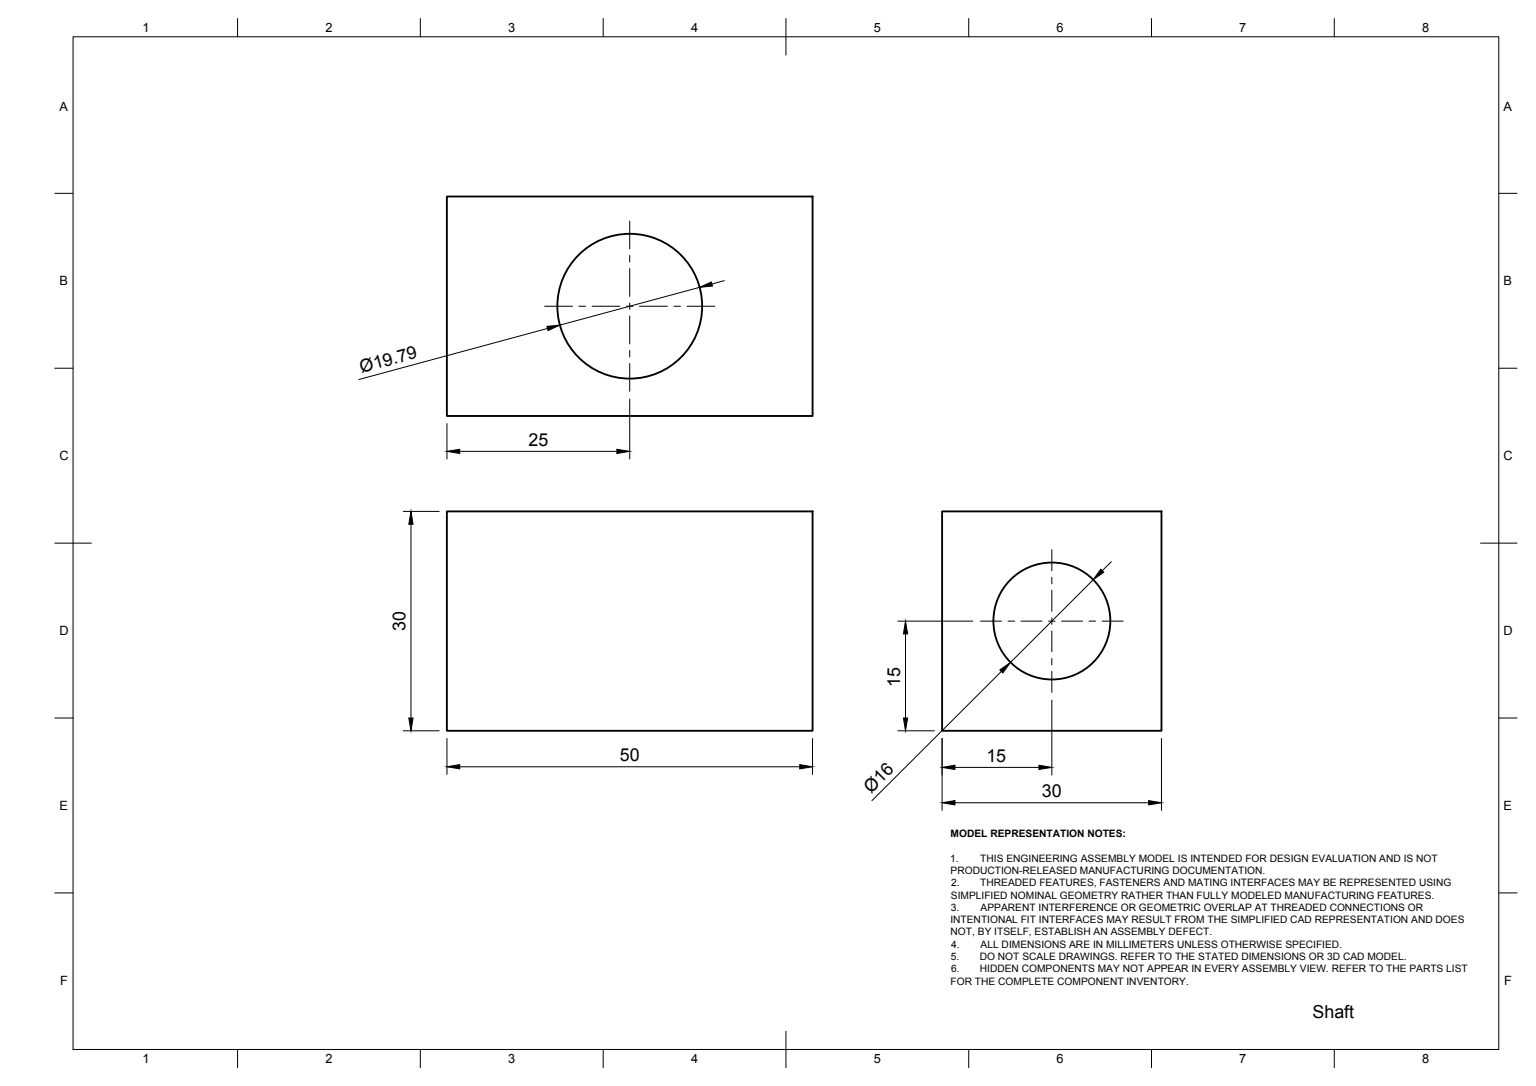
ISO-10303-21;
HEADER;
/* Generated by software containing ST-Developer
 * from STEP Tools, Inc. (www.steptools.com) 
 */

FILE_DESCRIPTION(
/* description */ (''),
/* implementation_level */ '2;1');

FILE_NAME(
/* name */ 'Shaft.step',
/* time_stamp */ '2026-10-05T19:45:59-07:00',
/* author */ (''),
/* organization */ (''),
/* preprocessor_version */ 'ST-DEVELOPER v20.2',
/* originating_system */ 'Autodesk Translation Framework v15.15.0.0',
/* authorisation */ '');

FILE_SCHEMA (('AUTOMOTIVE_DESIGN { 1 0 10303 214 3 1 1 }'));
ENDSEC;

DATA;
#10=MECHANICAL_DESIGN_GEOMETRIC_PRESENTATION_REPRESENTATION('',(#96),#2462);
#52=B_SPLINE_CURVE_WITH_KNOTS('',3,(#2172,#2173,#2174,#2175,#2176,#2177,
#2178,#2179,#2180,#2181,#2182,#2183,#2184,#2185,#2186,#2187,#2188,#2189,
#2190,#2191,#2192,#2193),.UNSPECIFIED.,.F.,.F.,(4,2,2,2,2,2,2,2,2,2,4),
(1.29528463060384,1.61362869954164,1.93197276847945,2.26127101484344,2.42592013802544,
2.59056926120743,2.75521838438943,2.91986750757142,3.24916575393542,3.56750982287322,
3.88585389181102),.UNSPECIFIED.);
#53=B_SPLINE_CURVE_WITH_KNOTS('',3,(#2198,#2199,#2200,#2201,#2202,#2203,
#2204,#2205,#2206,#2207,#2208,#2209),.UNSPECIFIED.,.F.,.F.,(4,2,2,2,2,4),
(0.,0.164649123182026,0.329298246364052,0.658596492728105,0.976940561665974,
1.29528463060384),.UNSPECIFIED.);
#54=B_SPLINE_CURVE_WITH_KNOTS('',3,(#2210,#2211,#2212,#2213,#2214,#2215,
#2216,#2217,#2218,#2219,#2220,#2221),.UNSPECIFIED.,.F.,.F.,(4,2,2,2,2,4),
(3.88585389181102,4.20419796074889,4.52254202968676,4.85184027605081,5.01648939923284,
5.18113852241487),.UNSPECIFIED.);
#55=B_SPLINE_CURVE_WITH_KNOTS('',3,(#2223,#2224,#2225,#2226,#2227,#2228,
#2229,#2230,#2231,#2232,#2233,#2234,#2235,#2236,#2237,#2238,#2239,#2240,
#2241,#2242,#2243,#2244,#2245,#2246,#2247,#2248,#2249,#2250,#2251,#2252,
#2253,#2254,#2255,#2256,#2257,#2258,#2259,#2260,#2261,#2262,#2263,#2264),
 .UNSPECIFIED.,.T.,.F.,(4,2,2,2,2,2,2,2,2,2,2,2,2,2,2,2,2,2,2,2,4),(0.,
0.164649123182026,0.329298246364052,0.658596492728105,0.976940561665974,
1.29528463060384,1.61362869954165,1.93197276847945,2.26127101484344,2.42592013802544,
2.59056926120743,2.75521838438943,2.91986750757143,3.24916575393542,3.56750982287322,
3.88585389181102,4.20419796074889,4.52254202968676,4.85184027605081,5.01648939923284,
5.18113852241487),.UNSPECIFIED.);
#65=FACE_BOUND('',#295,.T.);
#66=FACE_BOUND('',#298,.T.);
#67=FACE_BOUND('',#302,.T.);
#68=FACE_BOUND('',#305,.T.);
#69=FACE_BOUND('',#307,.T.);
#78=SHAPE_REPRESENTATION_RELATIONSHIP('SRR','None',#2504,#87);
#87=ADVANCED_BREP_SHAPE_REPRESENTATION('',(#105),#2459);
#96=STYLED_ITEM('',(#2552),#105);
#105=MANIFOLD_SOLID_BREP('Body1',#1333);
#136=PLANE('',#1515);
#137=PLANE('',#1518);
#138=PLANE('',#1519);
#139=PLANE('',#1520);
#140=PLANE('',#1521);
#141=PLANE('',#1522);
#206=FACE_OUTER_BOUND('',#294,.T.);
#207=FACE_OUTER_BOUND('',#296,.T.);
#208=FACE_OUTER_BOUND('',#297,.T.);
#209=FACE_OUTER_BOUND('',#299,.T.);
#210=FACE_OUTER_BOUND('',#300,.T.);
#211=FACE_OUTER_BOUND('',#301,.T.);
#212=FACE_OUTER_BOUND('',#303,.T.);
#213=FACE_OUTER_BOUND('',#304,.T.);
#214=FACE_OUTER_BOUND('',#306,.T.);
#294=EDGE_LOOP('',(#1054,#1055,#1056,#1057,#1058,#1059,#1060,#1061,#1062));
#295=EDGE_LOOP('',(#1063));
#296=EDGE_LOOP('',(#1064,#1065,#1066,#1067,#1068,#1069));
#297=EDGE_LOOP('',(#1070,#1071,#1072,#1073));
#298=EDGE_LOOP('',(#1074));
#299=EDGE_LOOP('',(#1075,#1076,#1077,#1078));
#300=EDGE_LOOP('',(#1079,#1080,#1081,#1082));
#301=EDGE_LOOP('',(#1083,#1084,#1085,#1086));
#302=EDGE_LOOP('',(#1087));
#303=EDGE_LOOP('',(#1088,#1089,#1090,#1091));
#304=EDGE_LOOP('',(#1092,#1093,#1094,#1095));
#305=EDGE_LOOP('',(#1096));
#306=EDGE_LOOP('',(#1097,#1098,#1099,#1100));
#307=EDGE_LOOP('',(#1101));
#395=LINE('',#2170,#514);
#396=LINE('',#2195,#515);
#397=LINE('',#2268,#516);
#398=LINE('',#2272,#517);
#399=LINE('',#2274,#518);
#400=LINE('',#2276,#519);
#401=LINE('',#2277,#520);
#402=LINE('',#2280,#521);
#403=LINE('',#2284,#522);
#404=LINE('',#2286,#523);
#405=LINE('',#2287,#524);
#406=LINE('',#2290,#525);
#407=LINE('',#2291,#526);
#408=LINE('',#2294,#527);
#409=LINE('',#2295,#528);
#410=LINE('',#2297,#529);
#514=VECTOR('',#1786,9.89525);
#515=VECTOR('',#1787,9.89525);
#516=VECTOR('',#1794,8.);
#517=VECTOR('',#1797,10.);
#518=VECTOR('',#1798,10.);
#519=VECTOR('',#1799,10.);
#520=VECTOR('',#1800,10.);
#521=VECTOR('',#1803,8.);
#522=VECTOR('',#1808,10.);
#523=VECTOR('',#1809,10.);
#524=VECTOR('',#1810,10.);
#525=VECTOR('',#1813,10.);
#526=VECTOR('',#1814,10.);
#527=VECTOR('',#1817,10.);
#528=VECTOR('',#1818,10.);
#529=VECTOR('',#1821,10.);
#603=CIRCLE('',#1511,9.89525);
#604=CIRCLE('',#1512,9.89525);
#605=CIRCLE('',#1514,8.);
#606=CIRCLE('',#1517,8.);
#674=VERTEX_POINT('',#2167);
#675=VERTEX_POINT('',#2169);
#676=VERTEX_POINT('',#2171);
#677=VERTEX_POINT('',#2194);
#678=VERTEX_POINT('',#2197);
#679=VERTEX_POINT('',#2222);
#680=VERTEX_POINT('',#2266);
#681=VERTEX_POINT('',#2270);
#682=VERTEX_POINT('',#2271);
#683=VERTEX_POINT('',#2273);
#684=VERTEX_POINT('',#2275);
#685=VERTEX_POINT('',#2279);
#686=VERTEX_POINT('',#2283);
#687=VERTEX_POINT('',#2285);
#688=VERTEX_POINT('',#2289);
#689=VERTEX_POINT('',#2293);
#808=EDGE_CURVE('',#674,#674,#603,.T.);
#809=EDGE_CURVE('',#674,#675,#395,.T.);
#810=EDGE_CURVE('',#676,#675,#52,.T.);
#811=EDGE_CURVE('',#676,#677,#396,.T.);
#812=EDGE_CURVE('',#677,#677,#604,.T.);
#813=EDGE_CURVE('',#678,#676,#53,.T.);
#814=EDGE_CURVE('',#675,#678,#54,.T.);
#815=EDGE_CURVE('',#679,#679,#55,.T.);
#816=EDGE_CURVE('',#680,#680,#605,.T.);
#817=EDGE_CURVE('',#680,#678,#397,.T.);
#818=EDGE_CURVE('',#681,#682,#398,.T.);
#819=EDGE_CURVE('',#682,#683,#399,.T.);
#820=EDGE_CURVE('',#683,#684,#400,.T.);
#821=EDGE_CURVE('',#684,#681,#401,.T.);
#822=EDGE_CURVE('',#679,#685,#402,.T.);
#823=EDGE_CURVE('',#685,#685,#606,.T.);
#824=EDGE_CURVE('',#686,#682,#403,.T.);
#825=EDGE_CURVE('',#687,#686,#404,.T.);
#826=EDGE_CURVE('',#683,#687,#405,.T.);
#827=EDGE_CURVE('',#688,#687,#406,.T.);
#828=EDGE_CURVE('',#684,#688,#407,.T.);
#829=EDGE_CURVE('',#689,#688,#408,.T.);
#830=EDGE_CURVE('',#681,#689,#409,.T.);
#831=EDGE_CURVE('',#686,#689,#410,.T.);
#1054=ORIENTED_EDGE('',*,*,#808,.F.);
#1055=ORIENTED_EDGE('',*,*,#809,.T.);
#1056=ORIENTED_EDGE('',*,*,#810,.F.);
#1057=ORIENTED_EDGE('',*,*,#811,.T.);
#1058=ORIENTED_EDGE('',*,*,#812,.F.);
#1059=ORIENTED_EDGE('',*,*,#811,.F.);
#1060=ORIENTED_EDGE('',*,*,#813,.F.);
#1061=ORIENTED_EDGE('',*,*,#814,.F.);
#1062=ORIENTED_EDGE('',*,*,#809,.F.);
#1063=ORIENTED_EDGE('',*,*,#815,.F.);
#1064=ORIENTED_EDGE('',*,*,#816,.F.);
#1065=ORIENTED_EDGE('',*,*,#817,.T.);
#1066=ORIENTED_EDGE('',*,*,#813,.T.);
#1067=ORIENTED_EDGE('',*,*,#810,.T.);
#1068=ORIENTED_EDGE('',*,*,#814,.T.);
#1069=ORIENTED_EDGE('',*,*,#817,.F.);
#1070=ORIENTED_EDGE('',*,*,#818,.T.);
#1071=ORIENTED_EDGE('',*,*,#819,.T.);
#1072=ORIENTED_EDGE('',*,*,#820,.T.);
#1073=ORIENTED_EDGE('',*,*,#821,.T.);
#1074=ORIENTED_EDGE('',*,*,#816,.T.);
#1075=ORIENTED_EDGE('',*,*,#815,.T.);
#1076=ORIENTED_EDGE('',*,*,#822,.T.);
#1077=ORIENTED_EDGE('',*,*,#823,.F.);
#1078=ORIENTED_EDGE('',*,*,#822,.F.);
#1079=ORIENTED_EDGE('',*,*,#824,.F.);
#1080=ORIENTED_EDGE('',*,*,#825,.F.);
#1081=ORIENTED_EDGE('',*,*,#826,.F.);
#1082=ORIENTED_EDGE('',*,*,#819,.F.);
#1083=ORIENTED_EDGE('',*,*,#826,.T.);
#1084=ORIENTED_EDGE('',*,*,#827,.F.);
#1085=ORIENTED_EDGE('',*,*,#828,.F.);
#1086=ORIENTED_EDGE('',*,*,#820,.F.);
#1087=ORIENTED_EDGE('',*,*,#812,.T.);
#1088=ORIENTED_EDGE('',*,*,#828,.T.);
#1089=ORIENTED_EDGE('',*,*,#829,.F.);
#1090=ORIENTED_EDGE('',*,*,#830,.F.);
#1091=ORIENTED_EDGE('',*,*,#821,.F.);
#1092=ORIENTED_EDGE('',*,*,#830,.T.);
#1093=ORIENTED_EDGE('',*,*,#831,.F.);
#1094=ORIENTED_EDGE('',*,*,#824,.T.);
#1095=ORIENTED_EDGE('',*,*,#818,.F.);
#1096=ORIENTED_EDGE('',*,*,#808,.T.);
#1097=ORIENTED_EDGE('',*,*,#831,.T.);
#1098=ORIENTED_EDGE('',*,*,#829,.T.);
#1099=ORIENTED_EDGE('',*,*,#827,.T.);
#1100=ORIENTED_EDGE('',*,*,#825,.T.);
#1101=ORIENTED_EDGE('',*,*,#823,.T.);
#1238=CYLINDRICAL_SURFACE('',#1510,9.89525);
#1239=CYLINDRICAL_SURFACE('',#1513,8.);
#1240=CYLINDRICAL_SURFACE('',#1516,8.);
#1288=ADVANCED_FACE('',(#206,#65),#1238,.F.);
#1289=ADVANCED_FACE('',(#207),#1239,.F.);
#1290=ADVANCED_FACE('',(#208,#66),#136,.F.);
#1291=ADVANCED_FACE('',(#209),#1240,.F.);
#1292=ADVANCED_FACE('',(#210),#137,.T.);
#1293=ADVANCED_FACE('',(#211,#67),#138,.T.);
#1294=ADVANCED_FACE('',(#212),#139,.T.);
#1295=ADVANCED_FACE('',(#213,#68),#140,.T.);
#1296=ADVANCED_FACE('',(#214,#69),#141,.T.);
#1333=CLOSED_SHELL('',(#1288,#1289,#1290,#1291,#1292,#1293,#1294,#1295,
#1296));
#1509=AXIS2_PLACEMENT_3D('',#2165,#1780,#1781);
#1510=AXIS2_PLACEMENT_3D('',#2166,#1782,#1783);
#1511=AXIS2_PLACEMENT_3D('',#2168,#1784,#1785);
#1512=AXIS2_PLACEMENT_3D('',#2196,#1788,#1789);
#1513=AXIS2_PLACEMENT_3D('',#2265,#1790,#1791);
#1514=AXIS2_PLACEMENT_3D('',#2267,#1792,#1793);
#1515=AXIS2_PLACEMENT_3D('',#2269,#1795,#1796);
#1516=AXIS2_PLACEMENT_3D('',#2278,#1801,#1802);
#1517=AXIS2_PLACEMENT_3D('',#2281,#1804,#1805);
#1518=AXIS2_PLACEMENT_3D('',#2282,#1806,#1807);
#1519=AXIS2_PLACEMENT_3D('',#2288,#1811,#1812);
#1520=AXIS2_PLACEMENT_3D('',#2292,#1815,#1816);
#1521=AXIS2_PLACEMENT_3D('',#2296,#1819,#1820);
#1522=AXIS2_PLACEMENT_3D('',#2298,#1822,#1823);
#1780=DIRECTION('axis',(0.,0.,1.));
#1781=DIRECTION('refdir',(1.,0.,0.));
#1782=DIRECTION('center_axis',(0.,0.,-1.));
#1783=DIRECTION('ref_axis',(-1.,0.,0.));
#1784=DIRECTION('center_axis',(0.,0.,-1.));
#1785=DIRECTION('ref_axis',(-1.,0.,0.));
#1786=DIRECTION('',(0.,0.,-1.));
#1787=DIRECTION('',(0.,0.,-1.));
#1788=DIRECTION('center_axis',(0.,7.40148683083438E-17,1.));
#1789=DIRECTION('ref_axis',(-1.,0.,0.));
#1790=DIRECTION('center_axis',(-1.,0.,0.));
#1791=DIRECTION('ref_axis',(0.,-1.,0.));
#1792=DIRECTION('center_axis',(-1.,0.,0.));
#1793=DIRECTION('ref_axis',(0.,-1.,0.));
#1794=DIRECTION('',(-1.,0.,0.));
#1795=DIRECTION('center_axis',(-1.,0.,0.));
#1796=DIRECTION('ref_axis',(0.,-1.,0.));
#1797=DIRECTION('',(0.,-1.,0.));
#1798=DIRECTION('',(0.,0.,-1.));
#1799=DIRECTION('',(0.,1.,-7.40148683083438E-17));
#1800=DIRECTION('',(0.,0.,1.));
#1801=DIRECTION('center_axis',(-1.,0.,0.));
#1802=DIRECTION('ref_axis',(0.,-1.,0.));
#1803=DIRECTION('',(-1.,0.,0.));
#1804=DIRECTION('center_axis',(1.,0.,0.));
#1805=DIRECTION('ref_axis',(0.,-1.,0.));
#1806=DIRECTION('center_axis',(0.,-1.,0.));
#1807=DIRECTION('ref_axis',(0.,0.,1.));
#1808=DIRECTION('',(1.,0.,0.));
#1809=DIRECTION('',(0.,0.,1.));
#1810=DIRECTION('',(-1.,0.,0.));
#1811=DIRECTION('center_axis',(0.,-7.40148683083438E-17,-1.));
#1812=DIRECTION('ref_axis',(0.,-1.,7.40148683083438E-17));
#1813=DIRECTION('',(0.,-1.,7.40148683083438E-17));
#1814=DIRECTION('',(-1.,0.,0.));
#1815=DIRECTION('center_axis',(0.,1.,0.));
#1816=DIRECTION('ref_axis',(0.,0.,-1.));
#1817=DIRECTION('',(0.,0.,-1.));
#1818=DIRECTION('',(-1.,0.,0.));
#1819=DIRECTION('center_axis',(0.,0.,1.));
#1820=DIRECTION('ref_axis',(0.,1.,0.));
#1821=DIRECTION('',(0.,1.,0.));
#1822=DIRECTION('center_axis',(-1.,0.,0.));
#1823=DIRECTION('ref_axis',(0.,-1.,0.));
#2165=CARTESIAN_POINT('',(0.,0.,0.));
#2166=CARTESIAN_POINT('Origin',(152.4,-2.52242671194836E-12,14.9999999999958));
#2167=CARTESIAN_POINT('',(162.29525,-2.52121489332443E-12,14.9999999999958));
#2168=CARTESIAN_POINT('Origin',(152.4,-2.52242671194836E-12,14.9999999999958));
#2169=CARTESIAN_POINT('',(162.29525,-1.26161109846903E-12,8.));
#2170=CARTESIAN_POINT('',(162.29525,-2.52363853057229E-12,14.9999999999958));
#2171=CARTESIAN_POINT('',(162.29525,-1.26119476483479E-12,-8.));
#2172=CARTESIAN_POINT('Ctrl Pts',(162.29525,1.66533453693773E-15,-8.));
#2173=CARTESIAN_POINT('Ctrl Pts',(162.29525,-1.06114689645934,-8.));
#2174=CARTESIAN_POINT('Ctrl Pts',(162.112073508216,-2.15862639679729,-7.77661292309447));
#2175=CARTESIAN_POINT('Ctrl Pts',(161.456447542343,-4.11883390373875,-6.9405026969991));
#2176=CARTESIAN_POINT('Ctrl Pts',(160.987841858536,-4.9837667164534,-6.32994178253133));
#2177=CARTESIAN_POINT('Ctrl Pts',(160.033751169964,-6.35310263577037,-4.96060586321443));
#2178=CARTESIAN_POINT('Ctrl Pts',(159.469158415985,-6.95125183484192,-4.09614535763875));
#2179=CARTESIAN_POINT('Ctrl Pts',(158.784045152537,-7.56664871511797,-2.64960450672535));
#2180=CARTESIAN_POINT('Ctrl Pts',(158.584436338924,-7.7265896208107,-2.14179168027124));
#2181=CARTESIAN_POINT('Ctrl Pts',(158.303524359677,-7.94328901302828,-1.09161265583592));
#2182=CARTESIAN_POINT('Ctrl Pts',(158.223742144235,-8.,-0.548830410606655));
#2183=CARTESIAN_POINT('Ctrl Pts',(158.223742144235,-8.,0.548830410606653));
#2184=CARTESIAN_POINT('Ctrl Pts',(158.303524359677,-7.94328901302828,1.09161265583591));
#2185=CARTESIAN_POINT('Ctrl Pts',(158.584436338924,-7.7265896208107,2.14179168027124));
#2186=CARTESIAN_POINT('Ctrl Pts',(158.784045152537,-7.56664871511797,2.64960450672535));
#2187=CARTESIAN_POINT('Ctrl Pts',(159.469158415985,-6.95125183484192,4.09614535763875));
#2188=CARTESIAN_POINT('Ctrl Pts',(160.033751169964,-6.35310263577037,4.96060586321443));
#2189=CARTESIAN_POINT('Ctrl Pts',(160.987841858536,-4.98376671645341,6.32994178253132));
#2190=CARTESIAN_POINT('Ctrl Pts',(161.456447542343,-4.11883390373875,6.94050269699909));
#2191=CARTESIAN_POINT('Ctrl Pts',(162.112073508216,-2.15862639679729,7.77661292309447));
#2192=CARTESIAN_POINT('Ctrl Pts',(162.29525,-1.06114689645934,8.));
#2193=CARTESIAN_POINT('Ctrl Pts',(162.29525,-1.94289029309402E-15,8.));
#2194=CARTESIAN_POINT('',(162.29525,-2.52121489332443E-12,-15.0000000000042));
#2195=CARTESIAN_POINT('',(162.29525,-2.52363853057229E-12,14.9999999999958));
#2196=CARTESIAN_POINT('Origin',(152.4,-2.52242671194836E-12,-15.0000000000042));
#2197=CARTESIAN_POINT('',(158.223742144228,8.,-4.16333634234434E-16));
#2198=CARTESIAN_POINT('Ctrl Pts',(158.223742144228,8.,-4.16333634234434E-16));
#2199=CARTESIAN_POINT('Ctrl Pts',(158.223742144228,8.,-0.548830410606754));
#2200=CARTESIAN_POINT('Ctrl Pts',(158.30352435967,7.94328901302826,-1.09161265583602));
#2201=CARTESIAN_POINT('Ctrl Pts',(158.584436338918,7.72658962081068,-2.1417916802713));
#2202=CARTESIAN_POINT('Ctrl Pts',(158.784045152531,7.56664871511797,-2.64960450672535));
#2203=CARTESIAN_POINT('Ctrl Pts',(159.46915841598,6.951251834842,-4.09614535763859));
#2204=CARTESIAN_POINT('Ctrl Pts',(160.03375116996,6.35310263577055,-4.96060586321418));
#2205=CARTESIAN_POINT('Ctrl Pts',(160.987841858533,4.98376671645374,-6.32994178253105));
#2206=CARTESIAN_POINT('Ctrl Pts',(161.45644754234,4.11883390373914,-6.94050269699888));
#2207=CARTESIAN_POINT('Ctrl Pts',(162.112073508215,2.1586263967976,-7.77661292309439));
#2208=CARTESIAN_POINT('Ctrl Pts',(162.29525,1.06114689645957,-8.));
#2209=CARTESIAN_POINT('Ctrl Pts',(162.29525,1.52655665885959E-15,-8.));
#2210=CARTESIAN_POINT('Ctrl Pts',(162.29525,5.55111512312578E-16,8.));
#2211=CARTESIAN_POINT('Ctrl Pts',(162.29525,1.06114689645957,8.));
#2212=CARTESIAN_POINT('Ctrl Pts',(162.112073508215,2.1586263967976,7.77661292309439));
#2213=CARTESIAN_POINT('Ctrl Pts',(161.45644754234,4.11883390373913,6.94050269699888));
#2214=CARTESIAN_POINT('Ctrl Pts',(160.987841858533,4.98376671645374,6.32994178253105));
#2215=CARTESIAN_POINT('Ctrl Pts',(160.03375116996,6.35310263577055,4.96060586321418));
#2216=CARTESIAN_POINT('Ctrl Pts',(159.46915841598,6.951251834842,4.09614535763859));
#2217=CARTESIAN_POINT('Ctrl Pts',(158.784045152531,7.56664871511797,2.64960450672535));
#2218=CARTESIAN_POINT('Ctrl Pts',(158.584436338918,7.72658962081068,2.1417916802713));
#2219=CARTESIAN_POINT('Ctrl Pts',(158.30352435967,7.94328901302826,1.09161265583602));
#2220=CARTESIAN_POINT('Ctrl Pts',(158.223742144228,8.,0.548830410606755));
#2221=CARTESIAN_POINT('Ctrl Pts',(158.223742144228,8.,1.11022302462516E-15));
#2222=CARTESIAN_POINT('',(146.576257855772,8.,2.77555756156289E-16));
#2223=CARTESIAN_POINT('Ctrl Pts',(146.576257855772,8.,2.77555756156289E-16));
#2224=CARTESIAN_POINT('Ctrl Pts',(146.576257855772,8.,0.548830410606754));
#2225=CARTESIAN_POINT('Ctrl Pts',(146.49647564033,7.94328901302826,1.09161265583602));
#2226=CARTESIAN_POINT('Ctrl Pts',(146.215563661082,7.72658962081068,2.1417916802713));
#2227=CARTESIAN_POINT('Ctrl Pts',(146.015954847468,7.56664871511797,2.64960450672535));
#2228=CARTESIAN_POINT('Ctrl Pts',(145.33084158402,6.951251834842,4.09614535763859));
#2229=CARTESIAN_POINT('Ctrl Pts',(144.76624883004,6.35310263577055,4.96060586321418));
#2230=CARTESIAN_POINT('Ctrl Pts',(143.812158141467,4.98376671645374,6.32994178253105));
#2231=CARTESIAN_POINT('Ctrl Pts',(143.34355245766,4.11883390373914,6.94050269699888));
#2232=CARTESIAN_POINT('Ctrl Pts',(142.687926491785,2.15862639679761,7.77661292309439));
#2233=CARTESIAN_POINT('Ctrl Pts',(142.50475,1.06114689645956,8.));
#2234=CARTESIAN_POINT('Ctrl Pts',(142.50475,-1.06114689645934,8.));
#2235=CARTESIAN_POINT('Ctrl Pts',(142.687926491784,-2.15862639679729,7.77661292309447));
#2236=CARTESIAN_POINT('Ctrl Pts',(143.343552457657,-4.11883390373876,6.94050269699909));
#2237=CARTESIAN_POINT('Ctrl Pts',(143.812158141464,-4.98376671645341,6.32994178253132));
#2238=CARTESIAN_POINT('Ctrl Pts',(144.766248830036,-6.35310263577037,4.96060586321443));
#2239=CARTESIAN_POINT('Ctrl Pts',(145.330841584015,-6.95125183484192,4.09614535763875));
#2240=CARTESIAN_POINT('Ctrl Pts',(146.015954847463,-7.56664871511797,2.64960450672535));
#2241=CARTESIAN_POINT('Ctrl Pts',(146.215563661076,-7.7265896208107,2.14179168027124));
#2242=CARTESIAN_POINT('Ctrl Pts',(146.496475640323,-7.94328901302828,1.09161265583591));
#2243=CARTESIAN_POINT('Ctrl Pts',(146.576257855765,-8.,0.548830410606653));
#2244=CARTESIAN_POINT('Ctrl Pts',(146.576257855765,-8.,-0.548830410606655));
#2245=CARTESIAN_POINT('Ctrl Pts',(146.496475640323,-7.94328901302828,-1.09161265583592));
#2246=CARTESIAN_POINT('Ctrl Pts',(146.215563661076,-7.7265896208107,-2.14179168027124));
#2247=CARTESIAN_POINT('Ctrl Pts',(146.015954847463,-7.56664871511797,-2.64960450672535));
#2248=CARTESIAN_POINT('Ctrl Pts',(145.330841584015,-6.95125183484192,-4.09614535763875));
#2249=CARTESIAN_POINT('Ctrl Pts',(144.766248830036,-6.35310263577037,-4.96060586321443));
#2250=CARTESIAN_POINT('Ctrl Pts',(143.812158141464,-4.9837667164534,-6.32994178253133));
#2251=CARTESIAN_POINT('Ctrl Pts',(143.343552457657,-4.11883390373876,-6.94050269699909));
#2252=CARTESIAN_POINT('Ctrl Pts',(142.687926491784,-2.15862639679729,-7.77661292309447));
#2253=CARTESIAN_POINT('Ctrl Pts',(142.50475,-1.06114689645934,-8.));
#2254=CARTESIAN_POINT('Ctrl Pts',(142.50475,1.06114689645956,-8.));
#2255=CARTESIAN_POINT('Ctrl Pts',(142.687926491785,2.15862639679761,-7.77661292309439));
#2256=CARTESIAN_POINT('Ctrl Pts',(143.34355245766,4.11883390373914,-6.94050269699887));
#2257=CARTESIAN_POINT('Ctrl Pts',(143.812158141467,4.98376671645374,-6.32994178253105));
#2258=CARTESIAN_POINT('Ctrl Pts',(144.76624883004,6.35310263577055,-4.96060586321418));
#2259=CARTESIAN_POINT('Ctrl Pts',(145.33084158402,6.951251834842,-4.09614535763859));
#2260=CARTESIAN_POINT('Ctrl Pts',(146.015954847468,7.56664871511797,-2.64960450672535));
#2261=CARTESIAN_POINT('Ctrl Pts',(146.215563661082,7.72658962081068,-2.1417916802713));
#2262=CARTESIAN_POINT('Ctrl Pts',(146.49647564033,7.94328901302826,-1.09161265583602));
#2263=CARTESIAN_POINT('Ctrl Pts',(146.576257855772,8.,-0.54883041060675));
#2264=CARTESIAN_POINT('Ctrl Pts',(146.576257855772,8.,3.53883589099269E-15));
#2265=CARTESIAN_POINT('Origin',(152.4,0.,0.));
#2266=CARTESIAN_POINT('',(177.4,8.,-9.79717439317883E-16));
#2267=CARTESIAN_POINT('Origin',(177.4,0.,0.));
#2268=CARTESIAN_POINT('',(152.4,8.,-9.79717439317883E-16));
#2269=CARTESIAN_POINT('Origin',(177.4,-2.52686760404686E-12,-4.20552481728009E-12));
#2270=CARTESIAN_POINT('',(177.4,14.9999999999975,14.9999999999958));
#2271=CARTESIAN_POINT('',(177.4,-15.0000000000025,14.9999999999958));
#2272=CARTESIAN_POINT('',(177.4,14.9999999999975,14.9999999999958));
#2273=CARTESIAN_POINT('',(177.4,-15.0000000000025,-15.0000000000042));
#2274=CARTESIAN_POINT('',(177.4,-15.0000000000025,14.9999999999958));
#2275=CARTESIAN_POINT('',(177.4,14.9999999999975,-15.0000000000042));
#2276=CARTESIAN_POINT('',(177.4,-15.0000000000025,-15.0000000000042));
#2277=CARTESIAN_POINT('',(177.4,14.9999999999975,-15.0000000000042));
#2278=CARTESIAN_POINT('Origin',(152.4,0.,0.));
#2279=CARTESIAN_POINT('',(127.4,8.,-9.79717439317883E-16));
#2280=CARTESIAN_POINT('',(152.4,8.,-9.79717439317883E-16));
#2281=CARTESIAN_POINT('Origin',(127.4,0.,0.));
#2282=CARTESIAN_POINT('Origin',(152.4,-15.0000000000025,-15.0000000000042));
#2283=CARTESIAN_POINT('',(127.4,-15.0000000000025,14.9999999999958));
#2284=CARTESIAN_POINT('',(152.4,-15.0000000000025,14.9999999999958));
#2285=CARTESIAN_POINT('',(127.4,-15.0000000000025,-15.0000000000042));
#2286=CARTESIAN_POINT('',(127.4,-15.0000000000025,14.9999999999958));
#2287=CARTESIAN_POINT('',(152.4,-15.0000000000025,-15.0000000000042));
#2288=CARTESIAN_POINT('Origin',(152.4,14.9999999999975,-15.0000000000042));
#2289=CARTESIAN_POINT('',(127.4,14.9999999999975,-15.0000000000042));
#2290=CARTESIAN_POINT('',(127.4,-15.0000000000025,-15.0000000000042));
#2291=CARTESIAN_POINT('',(152.4,14.9999999999975,-15.0000000000042));
#2292=CARTESIAN_POINT('Origin',(152.4,14.9999999999975,14.9999999999958));
#2293=CARTESIAN_POINT('',(127.4,14.9999999999975,14.9999999999958));
#2294=CARTESIAN_POINT('',(127.4,14.9999999999975,-15.0000000000042));
#2295=CARTESIAN_POINT('',(152.4,14.9999999999975,14.9999999999958));
#2296=CARTESIAN_POINT('Origin',(152.4,-15.0000000000025,14.9999999999958));
#2297=CARTESIAN_POINT('',(127.4,14.9999999999975,14.9999999999958));
#2298=CARTESIAN_POINT('Origin',(127.4,-2.52686760404686E-12,-4.20552481728009E-12));
#2448=UNCERTAINTY_MEASURE_WITH_UNIT(LENGTH_MEASURE(0.01),#2463,
'DISTANCE_ACCURACY_VALUE',
'Maximum model space distance between geometric entities at asserted c
onnectivities');
#2451=UNCERTAINTY_MEASURE_WITH_UNIT(LENGTH_MEASURE(0.01),#2463,
'DISTANCE_ACCURACY_VALUE',
'Maximum model space distance between geometric entities at asserted c
onnectivities');
#2459=(
GEOMETRIC_REPRESENTATION_CONTEXT(3)
GLOBAL_UNCERTAINTY_ASSIGNED_CONTEXT((#2448))
GLOBAL_UNIT_ASSIGNED_CONTEXT((#2463,#2465,#2466))
REPRESENTATION_CONTEXT('','3D')
);
#2462=(
GEOMETRIC_REPRESENTATION_CONTEXT(3)
GLOBAL_UNCERTAINTY_ASSIGNED_CONTEXT((#2451))
GLOBAL_UNIT_ASSIGNED_CONTEXT((#2463,#2465,#2466))
REPRESENTATION_CONTEXT('','3D')
);
#2463=(
LENGTH_UNIT()
NAMED_UNIT(*)
SI_UNIT(.MILLI.,.METRE.)
);
#2465=(
NAMED_UNIT(*)
PLANE_ANGLE_UNIT()
SI_UNIT($,.RADIAN.)
);
#2466=(
NAMED_UNIT(*)
SI_UNIT($,.STERADIAN.)
SOLID_ANGLE_UNIT()
);
#2474=SHAPE_DEFINITION_REPRESENTATION(#2484,#2504);
#2484=PRODUCT_DEFINITION_SHAPE('',$,#2515);
#2504=SHAPE_REPRESENTATION('',(#1509),#2459);
#2507=PRODUCT_DEFINITION_CONTEXT('part definition',#2539,'design');
#2515=PRODUCT_DEFINITION('Shaft','Shaft',#2525,#2507);
#2525=PRODUCT_DEFINITION_FORMATION('',$,#2548);
#2539=APPLICATION_CONTEXT(
'Core Data for Automotive Mechanical Design Process');
#2540=PRODUCT_CONTEXT('part definition',#2539,'mechanical');
#2548=PRODUCT('Shaft','Shaft',$,(#2540));
#2552=PRESENTATION_STYLE_ASSIGNMENT((#2555));
#2555=SURFACE_STYLE_USAGE(.BOTH.,#2558);
#2558=SURFACE_SIDE_STYLE('',(#2561));
#2561=SURFACE_STYLE_FILL_AREA(#2564);
#2564=FILL_AREA_STYLE('Opaque(160,160,160)',(#2567));
#2567=FILL_AREA_STYLE_COLOUR('Opaque(160,160,160)',#2570);
#2570=COLOUR_RGB('Opaque(160,160,160)', 0.09019608, 0.27058824, 0.51372549);
ENDSEC;
END-ISO-10303-21;
